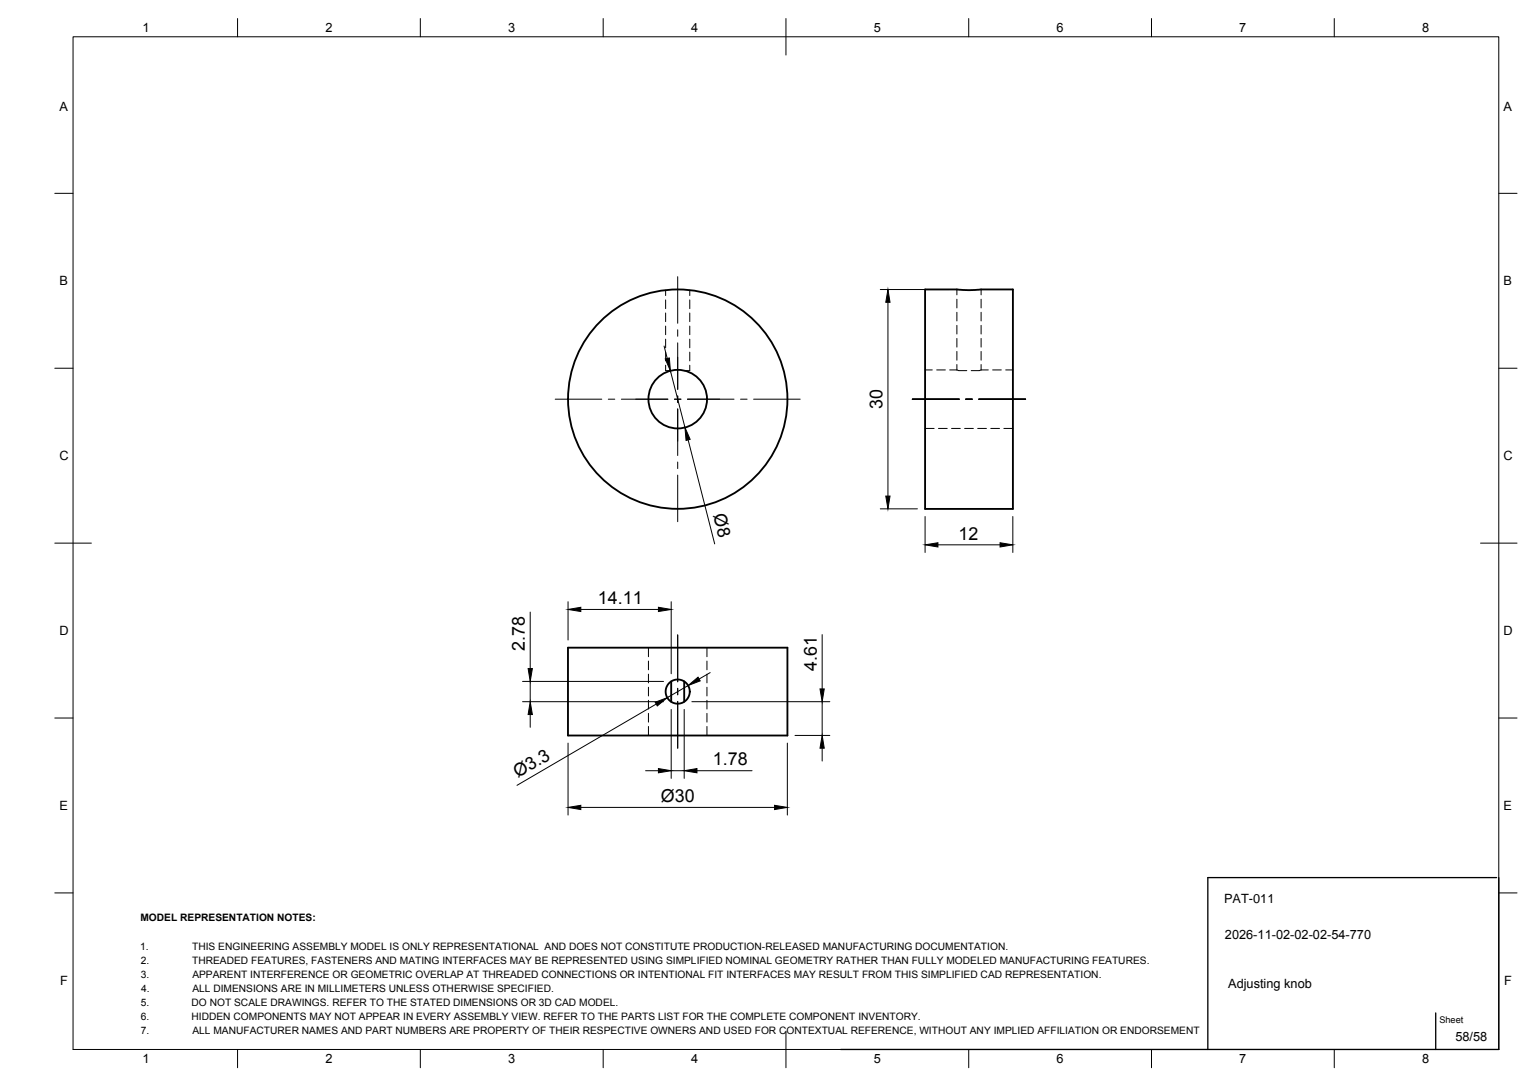
ISO-10303-21;
HEADER;
/* Generated by software containing ST-Developer
 * from STEP Tools, Inc. (www.steptools.com) 
 */

FILE_DESCRIPTION(
/* description */ ('Belt tension measurement rig'),
/* implementation_level */ '2;1');

FILE_NAME(
/* name */ 'Adjusting knob.step',
/* time_stamp */ '2026-10-28T03:24:44-07:00',
/* author */ (''),
/* organization */ (''),
/* preprocessor_version */ 'ST-DEVELOPER v20.2',
/* originating_system */ 'Autodesk Translation Framework v15.17.0.0',
/* authorisation */ '');

FILE_SCHEMA (('AUTOMOTIVE_DESIGN { 1 0 10303 214 3 1 1 }'));
ENDSEC;

DATA;
#10=MECHANICAL_DESIGN_GEOMETRIC_PRESENTATION_REPRESENTATION('',(#760),#23587);
#575=B_SPLINE_CURVE_WITH_KNOTS('',3,(#23279,#23280,#23281,#23282,#23283,
#23284),.UNSPECIFIED.,.F.,.F.,(4,2,4),(0.665271585430997,0.692803751398642,
0.755746158887618),.UNSPECIFIED.);
#576=B_SPLINE_CURVE_WITH_KNOTS('',3,(#23288,#23289,#23290,#23291,#23292,
#23293),.UNSPECIFIED.,.F.,.F.,(4,2,4),(0.251915386295873,0.31485779378485,
0.342389959752494),.UNSPECIFIED.);
#577=B_SPLINE_CURVE_WITH_KNOTS('',3,(#23294,#23295,#23296,#23297,#23298,
#23299),.UNSPECIFIED.,.F.,.F.,(4,2,4),(0.161440812839248,0.188972978806896,
0.251915386295873),.UNSPECIFIED.);
#578=B_SPLINE_CURVE_WITH_KNOTS('',3,(#23300,#23301,#23302,#23303,#23304,
#23305),.UNSPECIFIED.,.F.,.F.,(4,2,4),(0.755746158887618,0.818688566376595,
0.84622073234424),.UNSPECIFIED.);
#579=B_SPLINE_CURVE_WITH_KNOTS('',3,(#23309,#23310,#23311,#23312,#23313,
#23314,#23315,#23316,#23317,#23318),.UNSPECIFIED.,.F.,.F.,(4,2,2,2,4),(0.,
0.0622075173149514,0.124415034629903,0.186622241324509,0.248829448019115),
 .UNSPECIFIED.);
#580=B_SPLINE_CURVE_WITH_KNOTS('',3,(#23320,#23321,#23322,#23323,#23324,
#23325,#23326,#23327,#23328,#23329),.UNSPECIFIED.,.F.,.F.,(4,2,2,2,4),(0.746488344057344,
0.80869555075195,0.870902757446556,0.933110274761507,0.995317792076459),
 .UNSPECIFIED.);
#581=B_SPLINE_CURVE_WITH_KNOTS('',3,(#23330,#23331,#23332,#23333,#23334,
#23335,#23336,#23337,#23338,#23339,#23340,#23341,#23342,#23343,#23344,#23345,
#23346,#23347),.UNSPECIFIED.,.F.,.F.,(4,2,2,2,2,2,2,2,4),(0.248829448019115,
0.311036654713721,0.373243861408327,0.435451378723278,0.497658896038229,
0.559866413353181,0.622073930668132,0.684281137362738,0.746488344057344),
 .UNSPECIFIED.);
#635=SHAPE_REPRESENTATION_RELATIONSHIP('SRR','None',#23887,#690);
#690=ADVANCED_BREP_SHAPE_REPRESENTATION('',(#827),#23585);
#760=STYLED_ITEM('',(#24197),#827);
#827=MANIFOLD_SOLID_BREP('Body1',#12268);
#1034=FACE_BOUND('',#2952,.T.);
#1035=FACE_BOUND('',#2954,.T.);
#1339=PLANE('',#14449);
#1340=PLANE('',#14453);
#1341=PLANE('',#14460);
#1342=PLANE('',#14461);
#2037=FACE_OUTER_BOUND('',#2946,.T.);
#2038=FACE_OUTER_BOUND('',#2947,.T.);
#2039=FACE_OUTER_BOUND('',#2948,.T.);
#2040=FACE_OUTER_BOUND('',#2949,.T.);
#2041=FACE_OUTER_BOUND('',#2950,.T.);
#2042=FACE_OUTER_BOUND('',#2951,.T.);
#2043=FACE_OUTER_BOUND('',#2953,.T.);
#2946=EDGE_LOOP('',(#11068,#11069));
#2947=EDGE_LOOP('',(#11070,#11071,#11072,#11073,#11074,#11075,#11076,#11077,
#11078,#11079,#11080));
#2948=EDGE_LOOP('',(#11081,#11082));
#2949=EDGE_LOOP('',(#11083,#11084,#11085,#11086,#11087,#11088,#11089,#11090,
#11091,#11092,#11093,#11094));
#2950=EDGE_LOOP('',(#11095,#11096,#11097,#11098,#11099,#11100,#11101,#11102,
#11103));
#2951=EDGE_LOOP('',(#11104));
#2952=EDGE_LOOP('',(#11105));
#2953=EDGE_LOOP('',(#11106));
#2954=EDGE_LOOP('',(#11107));
#3691=LINE('',#23274,#4442);
#3692=LINE('',#23307,#4443);
#3693=LINE('',#23349,#4444);
#3694=LINE('',#23353,#4445);
#3695=LINE('',#23355,#4446);
#3696=LINE('',#23360,#4447);
#3697=LINE('',#23362,#4448);
#4442=VECTOR('',#18388,1.);
#4443=VECTOR('',#18395,0.165);
#4444=VECTOR('',#18398,1.);
#4445=VECTOR('',#18403,0.4);
#4446=VECTOR('',#18404,0.4);
#4447=VECTOR('',#18411,1.5);
#4448=VECTOR('',#18412,1.5);
#5228=CIRCLE('',#14450,0.165);
#5229=CIRCLE('',#14452,0.165);
#5230=CIRCLE('',#14455,0.4);
#5231=CIRCLE('',#14456,0.4);
#5232=CIRCLE('',#14458,1.5);
#5233=CIRCLE('',#14459,1.5);
#6299=VERTEX_POINT('',#23272);
#6300=VERTEX_POINT('',#23273);
#6301=VERTEX_POINT('',#23277);
#6302=VERTEX_POINT('',#23278);
#6303=VERTEX_POINT('',#23285);
#6304=VERTEX_POINT('',#23287);
#6305=VERTEX_POINT('',#23306);
#6306=VERTEX_POINT('',#23308);
#6307=VERTEX_POINT('',#23319);
#6308=VERTEX_POINT('',#23351);
#6309=VERTEX_POINT('',#23354);
#6310=VERTEX_POINT('',#23358);
#6311=VERTEX_POINT('',#23361);
#7893=EDGE_CURVE('',#6299,#6300,#3691,.T.);
#7894=EDGE_CURVE('',#6299,#6300,#5228,.T.);
#7895=EDGE_CURVE('',#6301,#6302,#575,.T.);
#7896=EDGE_CURVE('',#6303,#6301,#5229,.T.);
#7897=EDGE_CURVE('',#6304,#6303,#576,.T.);
#7898=EDGE_CURVE('',#6300,#6304,#577,.T.);
#7899=EDGE_CURVE('',#6302,#6299,#578,.T.);
#7900=EDGE_CURVE('',#6302,#6305,#3692,.T.);
#7901=EDGE_CURVE('',#6306,#6305,#579,.T.);
#7902=EDGE_CURVE('',#6307,#6306,#580,.T.);
#7903=EDGE_CURVE('',#6305,#6307,#581,.T.);
#7904=EDGE_CURVE('',#6303,#6301,#3693,.T.);
#7905=EDGE_CURVE('',#6308,#6308,#5230,.T.);
#7906=EDGE_CURVE('',#6308,#6304,#3694,.T.);
#7907=EDGE_CURVE('',#6302,#6309,#3695,.T.);
#7908=EDGE_CURVE('',#6309,#6309,#5231,.T.);
#7909=EDGE_CURVE('',#6310,#6310,#5232,.T.);
#7910=EDGE_CURVE('',#6310,#6307,#3696,.T.);
#7911=EDGE_CURVE('',#6305,#6311,#3697,.T.);
#7912=EDGE_CURVE('',#6311,#6311,#5233,.T.);
#11068=ORIENTED_EDGE('',*,*,#7893,.F.);
#11069=ORIENTED_EDGE('',*,*,#7894,.T.);
#11070=ORIENTED_EDGE('',*,*,#7895,.F.);
#11071=ORIENTED_EDGE('',*,*,#7896,.F.);
#11072=ORIENTED_EDGE('',*,*,#7897,.F.);
#11073=ORIENTED_EDGE('',*,*,#7898,.F.);
#11074=ORIENTED_EDGE('',*,*,#7894,.F.);
#11075=ORIENTED_EDGE('',*,*,#7899,.F.);
#11076=ORIENTED_EDGE('',*,*,#7900,.T.);
#11077=ORIENTED_EDGE('',*,*,#7901,.F.);
#11078=ORIENTED_EDGE('',*,*,#7902,.F.);
#11079=ORIENTED_EDGE('',*,*,#7903,.F.);
#11080=ORIENTED_EDGE('',*,*,#7900,.F.);
#11081=ORIENTED_EDGE('',*,*,#7904,.F.);
#11082=ORIENTED_EDGE('',*,*,#7896,.T.);
#11083=ORIENTED_EDGE('',*,*,#7905,.F.);
#11084=ORIENTED_EDGE('',*,*,#7906,.T.);
#11085=ORIENTED_EDGE('',*,*,#7897,.T.);
#11086=ORIENTED_EDGE('',*,*,#7904,.T.);
#11087=ORIENTED_EDGE('',*,*,#7895,.T.);
#11088=ORIENTED_EDGE('',*,*,#7907,.T.);
#11089=ORIENTED_EDGE('',*,*,#7908,.T.);
#11090=ORIENTED_EDGE('',*,*,#7907,.F.);
#11091=ORIENTED_EDGE('',*,*,#7899,.T.);
#11092=ORIENTED_EDGE('',*,*,#7893,.T.);
#11093=ORIENTED_EDGE('',*,*,#7898,.T.);
#11094=ORIENTED_EDGE('',*,*,#7906,.F.);
#11095=ORIENTED_EDGE('',*,*,#7909,.F.);
#11096=ORIENTED_EDGE('',*,*,#7910,.T.);
#11097=ORIENTED_EDGE('',*,*,#7902,.T.);
#11098=ORIENTED_EDGE('',*,*,#7901,.T.);
#11099=ORIENTED_EDGE('',*,*,#7911,.T.);
#11100=ORIENTED_EDGE('',*,*,#7912,.T.);
#11101=ORIENTED_EDGE('',*,*,#7911,.F.);
#11102=ORIENTED_EDGE('',*,*,#7903,.T.);
#11103=ORIENTED_EDGE('',*,*,#7910,.F.);
#11104=ORIENTED_EDGE('',*,*,#7909,.T.);
#11105=ORIENTED_EDGE('',*,*,#7905,.T.);
#11106=ORIENTED_EDGE('',*,*,#7912,.F.);
#11107=ORIENTED_EDGE('',*,*,#7908,.F.);
#11489=CYLINDRICAL_SURFACE('',#14451,0.165);
#11490=CYLINDRICAL_SURFACE('',#14454,0.4);
#11491=CYLINDRICAL_SURFACE('',#14457,1.5);
#12178=ADVANCED_FACE('',(#2037),#1339,.T.);
#12179=ADVANCED_FACE('',(#2038),#11489,.F.);
#12180=ADVANCED_FACE('',(#2039),#1340,.T.);
#12181=ADVANCED_FACE('',(#2040),#11490,.F.);
#12182=ADVANCED_FACE('',(#2041),#11491,.T.);
#12183=ADVANCED_FACE('',(#2042,#1034),#1341,.T.);
#12184=ADVANCED_FACE('',(#2043,#1035),#1342,.F.);
#12268=CLOSED_SHELL('',(#12178,#12179,#12180,#12181,#12182,#12183,#12184));
#14448=AXIS2_PLACEMENT_3D('',#23270,#18384,#18385);
#14449=AXIS2_PLACEMENT_3D('',#23271,#18386,#18387);
#14450=AXIS2_PLACEMENT_3D('',#23275,#18389,#18390);
#14451=AXIS2_PLACEMENT_3D('',#23276,#18391,#18392);
#14452=AXIS2_PLACEMENT_3D('',#23286,#18393,#18394);
#14453=AXIS2_PLACEMENT_3D('',#23348,#18396,#18397);
#14454=AXIS2_PLACEMENT_3D('',#23350,#18399,#18400);
#14455=AXIS2_PLACEMENT_3D('',#23352,#18401,#18402);
#14456=AXIS2_PLACEMENT_3D('',#23356,#18405,#18406);
#14457=AXIS2_PLACEMENT_3D('',#23357,#18407,#18408);
#14458=AXIS2_PLACEMENT_3D('',#23359,#18409,#18410);
#14459=AXIS2_PLACEMENT_3D('',#23363,#18413,#18414);
#14460=AXIS2_PLACEMENT_3D('',#23364,#18415,#18416);
#14461=AXIS2_PLACEMENT_3D('',#23365,#18417,#18418);
#18384=DIRECTION('axis',(0.,0.,1.));
#18385=DIRECTION('refdir',(1.,0.,0.));
#18386=DIRECTION('center_axis',(0.,0.,1.));
#18387=DIRECTION('ref_axis',(1.,0.,0.));
#18388=DIRECTION('',(1.,0.,0.));
#18389=DIRECTION('center_axis',(0.,0.,1.));
#18390=DIRECTION('ref_axis',(1.,0.,0.));
#18391=DIRECTION('center_axis',(0.,0.,1.));
#18392=DIRECTION('ref_axis',(1.,0.,0.));
#18393=DIRECTION('center_axis',(0.,0.,1.));
#18394=DIRECTION('ref_axis',(1.,0.,0.));
#18395=DIRECTION('',(0.,0.,1.));
#18396=DIRECTION('center_axis',(0.,0.,1.));
#18397=DIRECTION('ref_axis',(1.,0.,0.));
#18398=DIRECTION('',(-1.,0.,0.));
#18399=DIRECTION('center_axis',(1.,0.,0.));
#18400=DIRECTION('ref_axis',(0.,0.,-1.));
#18401=DIRECTION('center_axis',(-1.,0.,0.));
#18402=DIRECTION('ref_axis',(0.,0.,-1.));
#18403=DIRECTION('',(-1.,0.,0.));
#18404=DIRECTION('',(-1.,0.,0.));
#18405=DIRECTION('center_axis',(-1.,0.,0.));
#18406=DIRECTION('ref_axis',(0.,0.,-1.));
#18407=DIRECTION('center_axis',(1.,0.,0.));
#18408=DIRECTION('ref_axis',(0.,0.,-1.));
#18409=DIRECTION('center_axis',(1.,0.,0.));
#18410=DIRECTION('ref_axis',(0.,0.,-1.));
#18411=DIRECTION('',(-1.,0.,0.));
#18412=DIRECTION('',(-1.,0.,0.));
#18413=DIRECTION('center_axis',(1.,0.,0.));
#18414=DIRECTION('ref_axis',(0.,0.,-1.));
#18415=DIRECTION('center_axis',(1.,0.,0.));
#18416=DIRECTION('ref_axis',(0.,0.,-1.));
#18417=DIRECTION('center_axis',(1.,0.,0.));
#18418=DIRECTION('ref_axis',(0.,0.,-1.));
#23270=CARTESIAN_POINT('',(0.,0.,0.));
#23271=CARTESIAN_POINT('Origin',(0.4,11.,4.89));
#23272=CARTESIAN_POINT('',(0.260985612255421,10.9111180558268,4.89));
#23273=CARTESIAN_POINT('',(0.539014387744579,10.9111180558268,4.89));
#23274=CARTESIAN_POINT('',(-0.2,10.9111180558268,4.89));
#23275=CARTESIAN_POINT('Origin',(0.4,11.,4.89));
#23276=CARTESIAN_POINT('Origin',(0.4,11.,4.89));
#23277=CARTESIAN_POINT('',(0.260985612255421,11.0888819441732,4.89));
#23278=CARTESIAN_POINT('',(0.235,11.,4.9));
#23279=CARTESIAN_POINT('Ctrl Pts',(0.260985612255421,11.0888819441732,4.89));
#23280=CARTESIAN_POINT('Ctrl Pts',(0.255879904539473,11.08089644342,4.89181991495419));
#23281=CARTESIAN_POINT('Ctrl Pts',(0.251403608139787,11.0723643333024,4.89350251788328));
#23282=CARTESIAN_POINT('Ctrl Pts',(0.239243775830271,11.0431949313469,4.89819171553211));
#23283=CARTESIAN_POINT('Ctrl Pts',(0.235,11.0209808024963,4.9));
#23284=CARTESIAN_POINT('Ctrl Pts',(0.235,11.,4.9));
#23285=CARTESIAN_POINT('',(0.539014387744579,11.0888819441732,4.89));
#23286=CARTESIAN_POINT('Origin',(0.4,11.,4.89));
#23287=CARTESIAN_POINT('',(0.565,11.,4.9));
#23288=CARTESIAN_POINT('Ctrl Pts',(0.565,11.,4.9));
#23289=CARTESIAN_POINT('Ctrl Pts',(0.565,11.0209808024963,4.9));
#23290=CARTESIAN_POINT('Ctrl Pts',(0.560756224169729,11.0431949313469,4.89819171553211));
#23291=CARTESIAN_POINT('Ctrl Pts',(0.548596391860213,11.0723643333024,4.89350251788328));
#23292=CARTESIAN_POINT('Ctrl Pts',(0.544120095460527,11.08089644342,4.89181991495419));
#23293=CARTESIAN_POINT('Ctrl Pts',(0.539014387744579,11.0888819441732,4.89));
#23294=CARTESIAN_POINT('Ctrl Pts',(0.539014387744579,10.9111180558268,4.89));
#23295=CARTESIAN_POINT('Ctrl Pts',(0.544120095460527,10.91910355658,4.89181991495419));
#23296=CARTESIAN_POINT('Ctrl Pts',(0.548596391860213,10.9276356666976,4.89350251788328));
#23297=CARTESIAN_POINT('Ctrl Pts',(0.560756224169729,10.9568050686531,4.89819171553211));
#23298=CARTESIAN_POINT('Ctrl Pts',(0.565,10.9790191975037,4.9));
#23299=CARTESIAN_POINT('Ctrl Pts',(0.565,11.,4.9));
#23300=CARTESIAN_POINT('Ctrl Pts',(0.235,11.,4.9));
#23301=CARTESIAN_POINT('Ctrl Pts',(0.235,10.9790191975037,4.9));
#23302=CARTESIAN_POINT('Ctrl Pts',(0.239243775830271,10.9568050686531,4.89819171553211));
#23303=CARTESIAN_POINT('Ctrl Pts',(0.251403608139787,10.9276356666976,4.89350251788328));
#23304=CARTESIAN_POINT('Ctrl Pts',(0.255879904539473,10.91910355658,4.89181991495419));
#23305=CARTESIAN_POINT('Ctrl Pts',(0.260985612255421,10.9111180558268,4.89));
#23306=CARTESIAN_POINT('',(0.235,11.,6.));
#23307=CARTESIAN_POINT('',(0.235,11.,4.89));
#23308=CARTESIAN_POINT('',(0.4,10.835,5.99089738077441));
#23309=CARTESIAN_POINT('Ctrl Pts',(0.4,10.835,5.99089738077441));
#23310=CARTESIAN_POINT('Ctrl Pts',(0.379264160895016,10.835,5.99089738077441));
#23311=CARTESIAN_POINT('Ctrl Pts',(0.35715772909914,10.8391475009749,5.99137458218466));
#23312=CARTESIAN_POINT('Ctrl Pts',(0.316510155068951,10.8559915528391,5.99309518705251));
#23313=CARTESIAN_POINT('Ctrl Pts',(0.297967572401872,10.8686871898066,5.99431341615514));
#23314=CARTESIAN_POINT('Ctrl Pts',(0.268687262909328,10.8979674992991,5.99659781052538));
#23315=CARTESIAN_POINT('Ctrl Pts',(0.255991568780354,10.9165101139013,5.99781281581157));
#23316=CARTESIAN_POINT('Ctrl Pts',(0.239147474615801,10.9571577954068,5.99952603771524));
#23317=CARTESIAN_POINT('Ctrl Pts',(0.235,10.9792642644351,6.));
#23318=CARTESIAN_POINT('Ctrl Pts',(0.235,11.,6.));
#23319=CARTESIAN_POINT('',(0.565,11.,6.));
#23320=CARTESIAN_POINT('Ctrl Pts',(0.565,11.,6.));
#23321=CARTESIAN_POINT('Ctrl Pts',(0.565,10.9792642644351,6.));
#23322=CARTESIAN_POINT('Ctrl Pts',(0.5608525253842,10.9571577954068,5.99952603771524));
#23323=CARTESIAN_POINT('Ctrl Pts',(0.544008431219647,10.9165101139013,5.99781281581157));
#23324=CARTESIAN_POINT('Ctrl Pts',(0.531312737090672,10.8979674992991,5.99659781052538));
#23325=CARTESIAN_POINT('Ctrl Pts',(0.502032427598128,10.8686871898066,5.99431341615514));
#23326=CARTESIAN_POINT('Ctrl Pts',(0.483489844931049,10.8559915528391,5.99309518705251));
#23327=CARTESIAN_POINT('Ctrl Pts',(0.44284227090086,10.8391475009749,5.99137458218466));
#23328=CARTESIAN_POINT('Ctrl Pts',(0.420735839104984,10.835,5.99089738077441));
#23329=CARTESIAN_POINT('Ctrl Pts',(0.4,10.835,5.99089738077441));
#23330=CARTESIAN_POINT('Ctrl Pts',(0.235,11.,6.));
#23331=CARTESIAN_POINT('Ctrl Pts',(0.235,11.0207357355649,6.));
#23332=CARTESIAN_POINT('Ctrl Pts',(0.2391474746158,11.0428422045932,5.99952603771524));
#23333=CARTESIAN_POINT('Ctrl Pts',(0.255991568780353,11.0834898860987,5.99781281581157));
#23334=CARTESIAN_POINT('Ctrl Pts',(0.268687262909328,11.1020325007009,5.99659781052538));
#23335=CARTESIAN_POINT('Ctrl Pts',(0.297967572401872,11.1313128101934,5.99431341615514));
#23336=CARTESIAN_POINT('Ctrl Pts',(0.316510155068951,11.1440084471609,5.99309518705251));
#23337=CARTESIAN_POINT('Ctrl Pts',(0.35715772909914,11.1608524990251,5.99137458218466));
#23338=CARTESIAN_POINT('Ctrl Pts',(0.379264160895016,11.165,5.99089738077441));
#23339=CARTESIAN_POINT('Ctrl Pts',(0.420735839104984,11.165,5.99089738077441));
#23340=CARTESIAN_POINT('Ctrl Pts',(0.44284227090086,11.1608524990251,5.99137458218466));
#23341=CARTESIAN_POINT('Ctrl Pts',(0.483489844931049,11.1440084471609,5.99309518705251));
#23342=CARTESIAN_POINT('Ctrl Pts',(0.502032427598128,11.1313128101934,5.99431341615514));
#23343=CARTESIAN_POINT('Ctrl Pts',(0.531312737090672,11.1020325007009,5.99659781052538));
#23344=CARTESIAN_POINT('Ctrl Pts',(0.544008431219647,11.0834898860987,5.99781281581157));
#23345=CARTESIAN_POINT('Ctrl Pts',(0.5608525253842,11.0428422045932,5.99952603771524));
#23346=CARTESIAN_POINT('Ctrl Pts',(0.565,11.0207357355649,6.));
#23347=CARTESIAN_POINT('Ctrl Pts',(0.565,11.,6.));
#23348=CARTESIAN_POINT('Origin',(0.4,11.,4.89));
#23349=CARTESIAN_POINT('',(-0.2,11.0888819441732,4.89));
#23350=CARTESIAN_POINT('Origin',(-0.2,11.,4.5));
#23351=CARTESIAN_POINT('',(1.,11.,4.9));
#23352=CARTESIAN_POINT('Origin',(1.,11.,4.5));
#23353=CARTESIAN_POINT('',(-0.2,11.,4.9));
#23354=CARTESIAN_POINT('',(-0.2,11.,4.9));
#23355=CARTESIAN_POINT('',(-0.2,11.,4.9));
#23356=CARTESIAN_POINT('Origin',(-0.2,11.,4.5));
#23357=CARTESIAN_POINT('Origin',(-0.2,11.,4.5));
#23358=CARTESIAN_POINT('',(1.,11.,6.));
#23359=CARTESIAN_POINT('Origin',(1.,11.,4.5));
#23360=CARTESIAN_POINT('',(-0.2,11.,6.));
#23361=CARTESIAN_POINT('',(-0.2,11.,6.));
#23362=CARTESIAN_POINT('',(-0.2,11.,6.));
#23363=CARTESIAN_POINT('Origin',(-0.2,11.,4.5));
#23364=CARTESIAN_POINT('Origin',(1.,11.,4.5));
#23365=CARTESIAN_POINT('Origin',(-0.2,11.,4.5));
#23520=UNCERTAINTY_MEASURE_WITH_UNIT(LENGTH_MEASURE(0.001),#23588,
'DISTANCE_ACCURACY_VALUE',
'Maximum model space distance between geometric entities at asserted c
onnectivities');
#23522=UNCERTAINTY_MEASURE_WITH_UNIT(LENGTH_MEASURE(0.001),#23588,
'DISTANCE_ACCURACY_VALUE',
'Maximum model space distance between geometric entities at asserted c
onnectivities');
#23585=(
GEOMETRIC_REPRESENTATION_CONTEXT(3)
GLOBAL_UNCERTAINTY_ASSIGNED_CONTEXT((#23520))
GLOBAL_UNIT_ASSIGNED_CONTEXT((#23588,#23590,#23591))
REPRESENTATION_CONTEXT('','3D')
);
#23587=(
GEOMETRIC_REPRESENTATION_CONTEXT(3)
GLOBAL_UNCERTAINTY_ASSIGNED_CONTEXT((#23522))
GLOBAL_UNIT_ASSIGNED_CONTEXT((#23588,#23590,#23591))
REPRESENTATION_CONTEXT('','3D')
);
#23588=(
LENGTH_UNIT()
NAMED_UNIT(*)
SI_UNIT(.CENTI.,.METRE.)
);
#23590=(
NAMED_UNIT(*)
PLANE_ANGLE_UNIT()
SI_UNIT($,.RADIAN.)
);
#23591=(
NAMED_UNIT(*)
SI_UNIT($,.STERADIAN.)
SOLID_ANGLE_UNIT()
);
#23654=SHAPE_DEFINITION_REPRESENTATION(#23785,#23887);
#23785=PRODUCT_DEFINITION_SHAPE('',$,#23952);
#23887=SHAPE_REPRESENTATION('',(#14448),#23585);
#23889=PRODUCT_DEFINITION_CONTEXT('part definition',#24083,'design');
#23952=PRODUCT_DEFINITION('Adjusting knob','Adjusting knob',#24016,#23889);
#24016=PRODUCT_DEFINITION_FORMATION('',$,#24147);
#24083=APPLICATION_CONTEXT(
'Core Data for Automotive Mechanical Design Process');
#24084=PRODUCT_CONTEXT('part definition',#24083,'mechanical');
#24147=PRODUCT('Adjusting knob','Adjusting knob','Adjusting knob',(#24084));
#24191=COLOUR_RGB('Light Blue',0.38,0.62,0.78);
#24192=FILL_AREA_STYLE_COLOUR('',#24191);
#24193=FILL_AREA_STYLE('',(#24192));
#24194=SURFACE_STYLE_FILL_AREA(#24193);
#24195=SURFACE_SIDE_STYLE('',(#24194));
#24196=SURFACE_STYLE_USAGE(.BOTH.,#24195);
#24197=PRESENTATION_STYLE_ASSIGNMENT((#24196));
ENDSEC;
END-ISO-10303-21;
